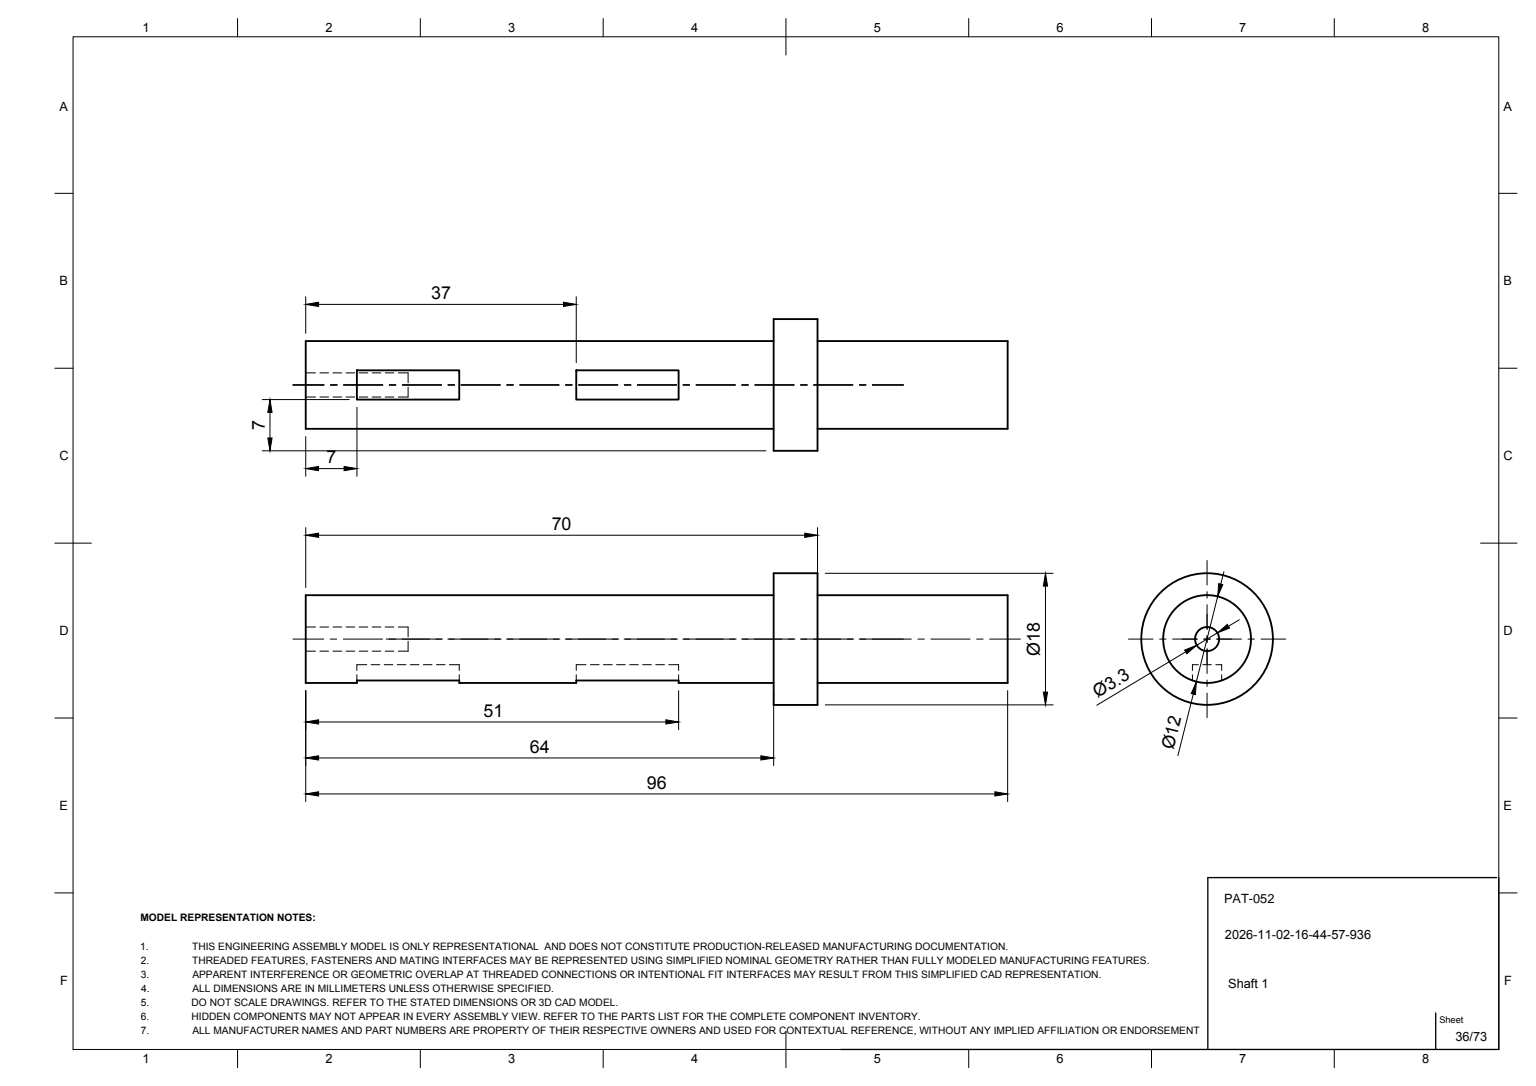
ISO-10303-21;
HEADER;
/* Generated by software containing ST-Developer
 * from STEP Tools, Inc. (www.steptools.com) 
 */

FILE_DESCRIPTION(
/* description */ ('Hand-crank gear train demonstrator'),
/* implementation_level */ '2;1');

FILE_NAME(
/* name */ 'Shaft 1.step',
/* time_stamp */ '2026-10-28T03:22:13-07:00',
/* author */ (''),
/* organization */ (''),
/* preprocessor_version */ 'ST-DEVELOPER v20.2',
/* originating_system */ 'Autodesk Translation Framework v15.17.0.0',
/* authorisation */ '');

FILE_SCHEMA (('AUTOMOTIVE_DESIGN { 1 0 10303 214 3 1 1 }'));
ENDSEC;

DATA;
#10=MECHANICAL_DESIGN_GEOMETRIC_PRESENTATION_REPRESENTATION('',(#1232),#62758);
#1089=SHAPE_REPRESENTATION_RELATIONSHIP('SRR','None',#63064,#1153);
#1153=ADVANCED_BREP_SHAPE_REPRESENTATION('',(#1308),#62718);
#1232=STYLED_ITEM('',(#63462),#1308);
#1308=MANIFOLD_SOLID_BREP('Body1',#16415);
#1542=FACE_BOUND('',#3696,.T.);
#1543=FACE_BOUND('',#3698,.T.);
#1544=FACE_BOUND('',#3702,.T.);
#1545=FACE_BOUND('',#3703,.T.);
#1546=FACE_BOUND('',#3705,.T.);
#1883=PLANE('',#17977);
#1884=PLANE('',#17978);
#1885=PLANE('',#17979);
#1886=PLANE('',#17981);
#1887=PLANE('',#17982);
#1888=PLANE('',#17983);
#1889=PLANE('',#17985);
#1890=PLANE('',#17986);
#1891=PLANE('',#17988);
#1892=PLANE('',#17989);
#1893=PLANE('',#17990);
#1894=PLANE('',#17992);
#1895=PLANE('',#17995);
#1896=PLANE('',#18003);
#1897=PLANE('',#18004);
#2547=FACE_OUTER_BOUND('',#3683,.T.);
#2548=FACE_OUTER_BOUND('',#3684,.T.);
#2549=FACE_OUTER_BOUND('',#3685,.T.);
#2550=FACE_OUTER_BOUND('',#3686,.T.);
#2551=FACE_OUTER_BOUND('',#3687,.T.);
#2552=FACE_OUTER_BOUND('',#3688,.T.);
#2553=FACE_OUTER_BOUND('',#3689,.T.);
#2554=FACE_OUTER_BOUND('',#3690,.T.);
#2555=FACE_OUTER_BOUND('',#3691,.T.);
#2556=FACE_OUTER_BOUND('',#3692,.T.);
#2557=FACE_OUTER_BOUND('',#3693,.T.);
#2558=FACE_OUTER_BOUND('',#3694,.T.);
#2559=FACE_OUTER_BOUND('',#3695,.T.);
#2560=FACE_OUTER_BOUND('',#3697,.T.);
#2561=FACE_OUTER_BOUND('',#3699,.T.);
#2562=FACE_OUTER_BOUND('',#3700,.T.);
#2563=FACE_OUTER_BOUND('',#3701,.T.);
#2564=FACE_OUTER_BOUND('',#3704,.T.);
#2565=FACE_OUTER_BOUND('',#3706,.T.);
#3683=EDGE_LOOP('',(#12709,#12710,#12711,#12712));
#3684=EDGE_LOOP('',(#12713));
#3685=EDGE_LOOP('',(#12714,#12715,#12716,#12717));
#3686=EDGE_LOOP('',(#12718,#12719,#12720,#12721));
#3687=EDGE_LOOP('',(#12722,#12723,#12724,#12725));
#3688=EDGE_LOOP('',(#12726,#12727,#12728,#12729));
#3689=EDGE_LOOP('',(#12730,#12731,#12732,#12733));
#3690=EDGE_LOOP('',(#12734,#12735,#12736,#12737));
#3691=EDGE_LOOP('',(#12738,#12739,#12740,#12741));
#3692=EDGE_LOOP('',(#12742,#12743,#12744,#12745));
#3693=EDGE_LOOP('',(#12746,#12747,#12748,#12749));
#3694=EDGE_LOOP('',(#12750,#12751,#12752,#12753));
#3695=EDGE_LOOP('',(#12754));
#3696=EDGE_LOOP('',(#12755));
#3697=EDGE_LOOP('',(#12756));
#3698=EDGE_LOOP('',(#12757));
#3699=EDGE_LOOP('',(#12758,#12759,#12760,#12761));
#3700=EDGE_LOOP('',(#12762,#12763,#12764,#12765));
#3701=EDGE_LOOP('',(#12766,#12767,#12768,#12769));
#3702=EDGE_LOOP('',(#12770,#12771,#12772,#12773));
#3703=EDGE_LOOP('',(#12774,#12775,#12776,#12777));
#3704=EDGE_LOOP('',(#12778));
#3705=EDGE_LOOP('',(#12779));
#3706=EDGE_LOOP('',(#12780));
#4843=LINE('',#25989,#5975);
#4844=LINE('',#25995,#5976);
#4845=LINE('',#25997,#5977);
#4846=LINE('',#25999,#5978);
#4847=LINE('',#26000,#5979);
#4848=LINE('',#26005,#5980);
#4849=LINE('',#26006,#5981);
#4850=LINE('',#26009,#5982);
#4851=LINE('',#26011,#5983);
#4852=LINE('',#26012,#5984);
#4853=LINE('',#26014,#5985);
#4854=LINE('',#26020,#5986);
#4855=LINE('',#26022,#5987);
#4856=LINE('',#26024,#5988);
#4857=LINE('',#26025,#5989);
#4858=LINE('',#26030,#5990);
#4859=LINE('',#26031,#5991);
#4860=LINE('',#26034,#5992);
#4861=LINE('',#26036,#5993);
#4862=LINE('',#26037,#5994);
#4863=LINE('',#26039,#5995);
#4864=LINE('',#26053,#5996);
#4865=LINE('',#26056,#5997);
#4866=LINE('',#26061,#5998);
#5975=VECTOR('',#21024,0.165);
#5976=VECTOR('',#21031,1.);
#5977=VECTOR('',#21032,1.);
#5978=VECTOR('',#21033,1.);
#5979=VECTOR('',#21034,1.);
#5980=VECTOR('',#21039,1.);
#5981=VECTOR('',#21040,1.);
#5982=VECTOR('',#21043,1.);
#5983=VECTOR('',#21044,1.);
#5984=VECTOR('',#21045,1.);
#5985=VECTOR('',#21048,1.);
#5986=VECTOR('',#21055,1.);
#5987=VECTOR('',#21056,1.);
#5988=VECTOR('',#21057,1.);
#5989=VECTOR('',#21058,1.);
#5990=VECTOR('',#21063,1.);
#5991=VECTOR('',#21064,1.);
#5992=VECTOR('',#21067,1.);
#5993=VECTOR('',#21068,1.);
#5994=VECTOR('',#21069,1.);
#5995=VECTOR('',#21072,1.);
#5996=VECTOR('',#21091,0.9);
#5997=VECTOR('',#21094,0.6);
#5998=VECTOR('',#21101,0.6);
#6898=CIRCLE('',#17975,0.165);
#6899=CIRCLE('',#17976,0.165);
#6900=CIRCLE('',#17980,0.6);
#6901=CIRCLE('',#17984,0.6);
#6902=CIRCLE('',#17987,0.6);
#6903=CIRCLE('',#17991,0.6);
#6904=CIRCLE('',#17993,0.9);
#6905=CIRCLE('',#17994,0.6);
#6906=CIRCLE('',#17996,0.9);
#6907=CIRCLE('',#17997,0.6);
#6908=CIRCLE('',#18000,0.6);
#6909=CIRCLE('',#18002,0.6);
#7851=VERTEX_POINT('',#25986);
#7852=VERTEX_POINT('',#25988);
#7853=VERTEX_POINT('',#25993);
#7854=VERTEX_POINT('',#25994);
#7855=VERTEX_POINT('',#25996);
#7856=VERTEX_POINT('',#25998);
#7857=VERTEX_POINT('',#26002);
#7858=VERTEX_POINT('',#26004);
#7859=VERTEX_POINT('',#26008);
#7860=VERTEX_POINT('',#26010);
#7861=VERTEX_POINT('',#26018);
#7862=VERTEX_POINT('',#26019);
#7863=VERTEX_POINT('',#26021);
#7864=VERTEX_POINT('',#26023);
#7865=VERTEX_POINT('',#26027);
#7866=VERTEX_POINT('',#26029);
#7867=VERTEX_POINT('',#26033);
#7868=VERTEX_POINT('',#26035);
#7869=VERTEX_POINT('',#26043);
#7870=VERTEX_POINT('',#26045);
#7871=VERTEX_POINT('',#26048);
#7872=VERTEX_POINT('',#26050);
#7873=VERTEX_POINT('',#26055);
#7874=VERTEX_POINT('',#26059);
#9606=EDGE_CURVE('',#7851,#7851,#6898,.T.);
#9607=EDGE_CURVE('',#7851,#7852,#4843,.T.);
#9608=EDGE_CURVE('',#7852,#7852,#6899,.T.);
#9609=EDGE_CURVE('',#7853,#7854,#4844,.T.);
#9610=EDGE_CURVE('',#7853,#7855,#4845,.T.);
#9611=EDGE_CURVE('',#7856,#7855,#4846,.T.);
#9612=EDGE_CURVE('',#7856,#7854,#4847,.T.);
#9613=EDGE_CURVE('',#7854,#7857,#6900,.T.);
#9614=EDGE_CURVE('',#7858,#7856,#4848,.T.);
#9615=EDGE_CURVE('',#7857,#7858,#4849,.T.);
#9616=EDGE_CURVE('',#7857,#7859,#4850,.T.);
#9617=EDGE_CURVE('',#7858,#7860,#4851,.T.);
#9618=EDGE_CURVE('',#7860,#7859,#4852,.T.);
#9619=EDGE_CURVE('',#7855,#7860,#4853,.T.);
#9620=EDGE_CURVE('',#7859,#7853,#6901,.T.);
#9621=EDGE_CURVE('',#7861,#7862,#4854,.T.);
#9622=EDGE_CURVE('',#7861,#7863,#4855,.T.);
#9623=EDGE_CURVE('',#7864,#7863,#4856,.T.);
#9624=EDGE_CURVE('',#7864,#7862,#4857,.T.);
#9625=EDGE_CURVE('',#7862,#7865,#6902,.T.);
#9626=EDGE_CURVE('',#7866,#7864,#4858,.T.);
#9627=EDGE_CURVE('',#7865,#7866,#4859,.T.);
#9628=EDGE_CURVE('',#7865,#7867,#4860,.T.);
#9629=EDGE_CURVE('',#7866,#7868,#4861,.T.);
#9630=EDGE_CURVE('',#7868,#7867,#4862,.T.);
#9631=EDGE_CURVE('',#7863,#7868,#4863,.T.);
#9632=EDGE_CURVE('',#7867,#7861,#6903,.T.);
#9633=EDGE_CURVE('',#7869,#7869,#6904,.T.);
#9634=EDGE_CURVE('',#7870,#7870,#6905,.T.);
#9635=EDGE_CURVE('',#7871,#7871,#6906,.T.);
#9636=EDGE_CURVE('',#7872,#7872,#6907,.T.);
#9637=EDGE_CURVE('',#7869,#7871,#4864,.T.);
#9638=EDGE_CURVE('',#7872,#7873,#4865,.T.);
#9639=EDGE_CURVE('',#7873,#7873,#6908,.T.);
#9640=EDGE_CURVE('',#7874,#7874,#6909,.T.);
#9641=EDGE_CURVE('',#7874,#7870,#4866,.T.);
#12709=ORIENTED_EDGE('',*,*,#9606,.F.);
#12710=ORIENTED_EDGE('',*,*,#9607,.T.);
#12711=ORIENTED_EDGE('',*,*,#9608,.F.);
#12712=ORIENTED_EDGE('',*,*,#9607,.F.);
#12713=ORIENTED_EDGE('',*,*,#9606,.T.);
#12714=ORIENTED_EDGE('',*,*,#9609,.F.);
#12715=ORIENTED_EDGE('',*,*,#9610,.T.);
#12716=ORIENTED_EDGE('',*,*,#9611,.F.);
#12717=ORIENTED_EDGE('',*,*,#9612,.T.);
#12718=ORIENTED_EDGE('',*,*,#9613,.F.);
#12719=ORIENTED_EDGE('',*,*,#9612,.F.);
#12720=ORIENTED_EDGE('',*,*,#9614,.F.);
#12721=ORIENTED_EDGE('',*,*,#9615,.F.);
#12722=ORIENTED_EDGE('',*,*,#9616,.F.);
#12723=ORIENTED_EDGE('',*,*,#9615,.T.);
#12724=ORIENTED_EDGE('',*,*,#9617,.T.);
#12725=ORIENTED_EDGE('',*,*,#9618,.T.);
#12726=ORIENTED_EDGE('',*,*,#9614,.T.);
#12727=ORIENTED_EDGE('',*,*,#9611,.T.);
#12728=ORIENTED_EDGE('',*,*,#9619,.T.);
#12729=ORIENTED_EDGE('',*,*,#9617,.F.);
#12730=ORIENTED_EDGE('',*,*,#9620,.F.);
#12731=ORIENTED_EDGE('',*,*,#9618,.F.);
#12732=ORIENTED_EDGE('',*,*,#9619,.F.);
#12733=ORIENTED_EDGE('',*,*,#9610,.F.);
#12734=ORIENTED_EDGE('',*,*,#9621,.F.);
#12735=ORIENTED_EDGE('',*,*,#9622,.T.);
#12736=ORIENTED_EDGE('',*,*,#9623,.F.);
#12737=ORIENTED_EDGE('',*,*,#9624,.T.);
#12738=ORIENTED_EDGE('',*,*,#9625,.F.);
#12739=ORIENTED_EDGE('',*,*,#9624,.F.);
#12740=ORIENTED_EDGE('',*,*,#9626,.F.);
#12741=ORIENTED_EDGE('',*,*,#9627,.F.);
#12742=ORIENTED_EDGE('',*,*,#9628,.F.);
#12743=ORIENTED_EDGE('',*,*,#9627,.T.);
#12744=ORIENTED_EDGE('',*,*,#9629,.T.);
#12745=ORIENTED_EDGE('',*,*,#9630,.T.);
#12746=ORIENTED_EDGE('',*,*,#9626,.T.);
#12747=ORIENTED_EDGE('',*,*,#9623,.T.);
#12748=ORIENTED_EDGE('',*,*,#9631,.T.);
#12749=ORIENTED_EDGE('',*,*,#9629,.F.);
#12750=ORIENTED_EDGE('',*,*,#9632,.F.);
#12751=ORIENTED_EDGE('',*,*,#9630,.F.);
#12752=ORIENTED_EDGE('',*,*,#9631,.F.);
#12753=ORIENTED_EDGE('',*,*,#9622,.F.);
#12754=ORIENTED_EDGE('',*,*,#9633,.T.);
#12755=ORIENTED_EDGE('',*,*,#9634,.F.);
#12756=ORIENTED_EDGE('',*,*,#9635,.F.);
#12757=ORIENTED_EDGE('',*,*,#9636,.F.);
#12758=ORIENTED_EDGE('',*,*,#9633,.F.);
#12759=ORIENTED_EDGE('',*,*,#9637,.T.);
#12760=ORIENTED_EDGE('',*,*,#9635,.T.);
#12761=ORIENTED_EDGE('',*,*,#9637,.F.);
#12762=ORIENTED_EDGE('',*,*,#9636,.T.);
#12763=ORIENTED_EDGE('',*,*,#9638,.T.);
#12764=ORIENTED_EDGE('',*,*,#9639,.T.);
#12765=ORIENTED_EDGE('',*,*,#9638,.F.);
#12766=ORIENTED_EDGE('',*,*,#9640,.F.);
#12767=ORIENTED_EDGE('',*,*,#9641,.T.);
#12768=ORIENTED_EDGE('',*,*,#9634,.T.);
#12769=ORIENTED_EDGE('',*,*,#9641,.F.);
#12770=ORIENTED_EDGE('',*,*,#9616,.T.);
#12771=ORIENTED_EDGE('',*,*,#9620,.T.);
#12772=ORIENTED_EDGE('',*,*,#9609,.T.);
#12773=ORIENTED_EDGE('',*,*,#9613,.T.);
#12774=ORIENTED_EDGE('',*,*,#9628,.T.);
#12775=ORIENTED_EDGE('',*,*,#9632,.T.);
#12776=ORIENTED_EDGE('',*,*,#9621,.T.);
#12777=ORIENTED_EDGE('',*,*,#9625,.T.);
#12778=ORIENTED_EDGE('',*,*,#9640,.T.);
#12779=ORIENTED_EDGE('',*,*,#9608,.T.);
#12780=ORIENTED_EDGE('',*,*,#9639,.F.);
#15290=CYLINDRICAL_SURFACE('',#17974,0.165);
#15291=CYLINDRICAL_SURFACE('',#17998,0.9);
#15292=CYLINDRICAL_SURFACE('',#17999,0.6);
#15293=CYLINDRICAL_SURFACE('',#18001,0.6);
#15857=ADVANCED_FACE('',(#2547),#15290,.F.);
#15858=ADVANCED_FACE('',(#2548),#1883,.T.);
#15859=ADVANCED_FACE('',(#2549),#1884,.F.);
#15860=ADVANCED_FACE('',(#2550),#1885,.T.);
#15861=ADVANCED_FACE('',(#2551),#1886,.F.);
#15862=ADVANCED_FACE('',(#2552),#1887,.F.);
#15863=ADVANCED_FACE('',(#2553),#1888,.F.);
#15864=ADVANCED_FACE('',(#2554),#1889,.F.);
#15865=ADVANCED_FACE('',(#2555),#1890,.T.);
#15866=ADVANCED_FACE('',(#2556),#1891,.F.);
#15867=ADVANCED_FACE('',(#2557),#1892,.F.);
#15868=ADVANCED_FACE('',(#2558),#1893,.F.);
#15869=ADVANCED_FACE('',(#2559,#1542),#1894,.T.);
#15870=ADVANCED_FACE('',(#2560,#1543),#1895,.F.);
#15871=ADVANCED_FACE('',(#2561),#15291,.T.);
#15872=ADVANCED_FACE('',(#2562),#15292,.T.);
#15873=ADVANCED_FACE('',(#2563,#1544,#1545),#15293,.T.);
#15874=ADVANCED_FACE('',(#2564,#1546),#1896,.T.);
#15875=ADVANCED_FACE('',(#2565),#1897,.F.);
#16415=CLOSED_SHELL('',(#15857,#15858,#15859,#15860,#15861,#15862,#15863,
#15864,#15865,#15866,#15867,#15868,#15869,#15870,#15871,#15872,#15873,#15874,
#15875));
#17973=AXIS2_PLACEMENT_3D('',#25984,#21018,#21019);
#17974=AXIS2_PLACEMENT_3D('',#25985,#21020,#21021);
#17975=AXIS2_PLACEMENT_3D('',#25987,#21022,#21023);
#17976=AXIS2_PLACEMENT_3D('',#25990,#21025,#21026);
#17977=AXIS2_PLACEMENT_3D('',#25991,#21027,#21028);
#17978=AXIS2_PLACEMENT_3D('',#25992,#21029,#21030);
#17979=AXIS2_PLACEMENT_3D('',#26001,#21035,#21036);
#17980=AXIS2_PLACEMENT_3D('',#26003,#21037,#21038);
#17981=AXIS2_PLACEMENT_3D('',#26007,#21041,#21042);
#17982=AXIS2_PLACEMENT_3D('',#26013,#21046,#21047);
#17983=AXIS2_PLACEMENT_3D('',#26015,#21049,#21050);
#17984=AXIS2_PLACEMENT_3D('',#26016,#21051,#21052);
#17985=AXIS2_PLACEMENT_3D('',#26017,#21053,#21054);
#17986=AXIS2_PLACEMENT_3D('',#26026,#21059,#21060);
#17987=AXIS2_PLACEMENT_3D('',#26028,#21061,#21062);
#17988=AXIS2_PLACEMENT_3D('',#26032,#21065,#21066);
#17989=AXIS2_PLACEMENT_3D('',#26038,#21070,#21071);
#17990=AXIS2_PLACEMENT_3D('',#26040,#21073,#21074);
#17991=AXIS2_PLACEMENT_3D('',#26041,#21075,#21076);
#17992=AXIS2_PLACEMENT_3D('',#26042,#21077,#21078);
#17993=AXIS2_PLACEMENT_3D('',#26044,#21079,#21080);
#17994=AXIS2_PLACEMENT_3D('',#26046,#21081,#21082);
#17995=AXIS2_PLACEMENT_3D('',#26047,#21083,#21084);
#17996=AXIS2_PLACEMENT_3D('',#26049,#21085,#21086);
#17997=AXIS2_PLACEMENT_3D('',#26051,#21087,#21088);
#17998=AXIS2_PLACEMENT_3D('',#26052,#21089,#21090);
#17999=AXIS2_PLACEMENT_3D('',#26054,#21092,#21093);
#18000=AXIS2_PLACEMENT_3D('',#26057,#21095,#21096);
#18001=AXIS2_PLACEMENT_3D('',#26058,#21097,#21098);
#18002=AXIS2_PLACEMENT_3D('',#26060,#21099,#21100);
#18003=AXIS2_PLACEMENT_3D('',#26062,#21102,#21103);
#18004=AXIS2_PLACEMENT_3D('',#26063,#21104,#21105);
#21018=DIRECTION('axis',(0.,0.,1.));
#21019=DIRECTION('refdir',(1.,0.,0.));
#21020=DIRECTION('center_axis',(0.,1.,0.));
#21021=DIRECTION('ref_axis',(1.,0.,0.));
#21022=DIRECTION('center_axis',(0.,1.,0.));
#21023=DIRECTION('ref_axis',(1.,0.,0.));
#21024=DIRECTION('',(0.,1.,0.));
#21025=DIRECTION('center_axis',(0.,-1.,0.));
#21026=DIRECTION('ref_axis',(1.,0.,0.));
#21027=DIRECTION('center_axis',(0.,1.,0.));
#21028=DIRECTION('ref_axis',(1.,0.,0.));
#21029=DIRECTION('center_axis',(-1.,0.,0.));
#21030=DIRECTION('ref_axis',(0.,0.,1.));
#21031=DIRECTION('',(0.,-1.,0.));
#21032=DIRECTION('',(0.,0.,1.));
#21033=DIRECTION('',(0.,1.,0.));
#21034=DIRECTION('',(0.,0.,-1.));
#21035=DIRECTION('center_axis',(0.,1.,0.));
#21036=DIRECTION('ref_axis',(1.,0.,0.));
#21037=DIRECTION('center_axis',(0.,-1.,0.));
#21038=DIRECTION('ref_axis',(1.,0.,0.));
#21039=DIRECTION('',(-1.,0.,0.));
#21040=DIRECTION('',(0.,0.,1.));
#21041=DIRECTION('center_axis',(1.,0.,0.));
#21042=DIRECTION('ref_axis',(0.,0.,-1.));
#21043=DIRECTION('',(0.,1.,0.));
#21044=DIRECTION('',(0.,1.,0.));
#21045=DIRECTION('',(0.,0.,-1.));
#21046=DIRECTION('center_axis',(0.,0.,1.));
#21047=DIRECTION('ref_axis',(1.,0.,0.));
#21048=DIRECTION('',(1.,0.,0.));
#21049=DIRECTION('center_axis',(0.,1.,0.));
#21050=DIRECTION('ref_axis',(0.,0.,1.));
#21051=DIRECTION('center_axis',(0.,1.,0.));
#21052=DIRECTION('ref_axis',(1.,0.,0.));
#21053=DIRECTION('center_axis',(-1.,0.,0.));
#21054=DIRECTION('ref_axis',(0.,0.,1.));
#21055=DIRECTION('',(0.,-1.,0.));
#21056=DIRECTION('',(0.,0.,1.));
#21057=DIRECTION('',(0.,1.,0.));
#21058=DIRECTION('',(0.,0.,-1.));
#21059=DIRECTION('center_axis',(0.,1.,0.));
#21060=DIRECTION('ref_axis',(1.,0.,0.));
#21061=DIRECTION('center_axis',(0.,-1.,0.));
#21062=DIRECTION('ref_axis',(1.,0.,0.));
#21063=DIRECTION('',(-1.,0.,0.));
#21064=DIRECTION('',(0.,0.,1.));
#21065=DIRECTION('center_axis',(1.,0.,0.));
#21066=DIRECTION('ref_axis',(0.,0.,-1.));
#21067=DIRECTION('',(0.,1.,0.));
#21068=DIRECTION('',(0.,1.,0.));
#21069=DIRECTION('',(0.,0.,-1.));
#21070=DIRECTION('center_axis',(0.,0.,1.));
#21071=DIRECTION('ref_axis',(1.,0.,0.));
#21072=DIRECTION('',(1.,0.,0.));
#21073=DIRECTION('center_axis',(0.,1.,0.));
#21074=DIRECTION('ref_axis',(0.,0.,1.));
#21075=DIRECTION('center_axis',(0.,1.,0.));
#21076=DIRECTION('ref_axis',(1.,0.,0.));
#21077=DIRECTION('center_axis',(0.,1.,0.));
#21078=DIRECTION('ref_axis',(1.,0.,0.));
#21079=DIRECTION('center_axis',(0.,1.,0.));
#21080=DIRECTION('ref_axis',(1.,0.,0.));
#21081=DIRECTION('center_axis',(0.,1.,0.));
#21082=DIRECTION('ref_axis',(1.,0.,0.));
#21083=DIRECTION('center_axis',(0.,1.,0.));
#21084=DIRECTION('ref_axis',(1.,0.,0.));
#21085=DIRECTION('center_axis',(0.,1.,0.));
#21086=DIRECTION('ref_axis',(1.,0.,0.));
#21087=DIRECTION('center_axis',(0.,-1.,0.));
#21088=DIRECTION('ref_axis',(1.,0.,0.));
#21089=DIRECTION('center_axis',(0.,1.,0.));
#21090=DIRECTION('ref_axis',(1.,0.,0.));
#21091=DIRECTION('',(0.,-1.,0.));
#21092=DIRECTION('center_axis',(0.,1.,0.));
#21093=DIRECTION('ref_axis',(1.,0.,0.));
#21094=DIRECTION('',(0.,-1.,0.));
#21095=DIRECTION('center_axis',(0.,1.,0.));
#21096=DIRECTION('ref_axis',(1.,0.,0.));
#21097=DIRECTION('center_axis',(0.,1.,0.));
#21098=DIRECTION('ref_axis',(1.,0.,0.));
#21099=DIRECTION('center_axis',(0.,1.,0.));
#21100=DIRECTION('ref_axis',(1.,0.,0.));
#21101=DIRECTION('',(0.,-1.,0.));
#21102=DIRECTION('center_axis',(0.,1.,0.));
#21103=DIRECTION('ref_axis',(1.,0.,0.));
#21104=DIRECTION('center_axis',(0.,1.,0.));
#21105=DIRECTION('ref_axis',(1.,0.,0.));
#25984=CARTESIAN_POINT('',(0.,0.,0.));
#25985=CARTESIAN_POINT('Origin',(0.,4.6,9.));
#25986=CARTESIAN_POINT('',(-0.165,4.6,9.));
#25987=CARTESIAN_POINT('Origin',(0.,4.6,9.));
#25988=CARTESIAN_POINT('',(-0.165,6.,9.));
#25989=CARTESIAN_POINT('',(-0.165,4.6,9.));
#25990=CARTESIAN_POINT('Origin',(0.,6.,9.));
#25991=CARTESIAN_POINT('Origin',(0.,4.6,9.));
#25992=CARTESIAN_POINT('Origin',(-0.2,3.9,8.3));
#25993=CARTESIAN_POINT('',(-0.2,5.3,8.43431457505076));
#25994=CARTESIAN_POINT('',(-0.2,3.9,8.43431457505076));
#25995=CARTESIAN_POINT('',(-0.2,-3.6,8.43431457505076));
#25996=CARTESIAN_POINT('',(-0.2,5.3,8.65));
#25997=CARTESIAN_POINT('',(-0.2,5.3,8.65));
#25998=CARTESIAN_POINT('',(-0.2,3.9,8.65));
#25999=CARTESIAN_POINT('',(-0.2,3.9,8.65));
#26000=CARTESIAN_POINT('',(-0.2,3.9,8.65));
#26001=CARTESIAN_POINT('Origin',(0.,3.9,8.475));
#26002=CARTESIAN_POINT('',(0.2,3.9,8.43431457505076));
#26003=CARTESIAN_POINT('Origin',(0.,3.9,9.));
#26004=CARTESIAN_POINT('',(0.2,3.9,8.65));
#26005=CARTESIAN_POINT('',(0.2,3.9,8.65));
#26006=CARTESIAN_POINT('',(0.2,3.9,8.3));
#26007=CARTESIAN_POINT('Origin',(0.2,3.9,8.65));
#26008=CARTESIAN_POINT('',(0.2,5.3,8.43431457505076));
#26009=CARTESIAN_POINT('',(0.2,-3.6,8.43431457505076));
#26010=CARTESIAN_POINT('',(0.2,5.3,8.65));
#26011=CARTESIAN_POINT('',(0.2,3.9,8.65));
#26012=CARTESIAN_POINT('',(0.2,5.3,8.3));
#26013=CARTESIAN_POINT('Origin',(-0.2,3.9,8.65));
#26014=CARTESIAN_POINT('',(0.2,5.3,8.65));
#26015=CARTESIAN_POINT('Origin',(0.,5.3,8.475));
#26016=CARTESIAN_POINT('Origin',(0.,5.3,9.));
#26017=CARTESIAN_POINT('Origin',(-0.2,0.9,7.8));
#26018=CARTESIAN_POINT('',(-0.2,2.3,8.43431457505076));
#26019=CARTESIAN_POINT('',(-0.2,0.9,8.43431457505076));
#26020=CARTESIAN_POINT('',(-0.2,-3.6,8.43431457505076));
#26021=CARTESIAN_POINT('',(-0.2,2.3,8.65));
#26022=CARTESIAN_POINT('',(-0.2,2.3,8.65));
#26023=CARTESIAN_POINT('',(-0.2,0.9,8.65));
#26024=CARTESIAN_POINT('',(-0.2,0.9,8.65));
#26025=CARTESIAN_POINT('',(-0.2,0.9,8.65));
#26026=CARTESIAN_POINT('Origin',(0.,0.9,8.225));
#26027=CARTESIAN_POINT('',(0.2,0.9,8.43431457505076));
#26028=CARTESIAN_POINT('Origin',(0.,0.9,9.));
#26029=CARTESIAN_POINT('',(0.2,0.9,8.65));
#26030=CARTESIAN_POINT('',(0.2,0.9,8.65));
#26031=CARTESIAN_POINT('',(0.2,0.9,7.8));
#26032=CARTESIAN_POINT('Origin',(0.2,0.9,8.65));
#26033=CARTESIAN_POINT('',(0.2,2.3,8.43431457505076));
#26034=CARTESIAN_POINT('',(0.2,-3.6,8.43431457505076));
#26035=CARTESIAN_POINT('',(0.2,2.3,8.65));
#26036=CARTESIAN_POINT('',(0.2,0.9,8.65));
#26037=CARTESIAN_POINT('',(0.2,2.3,7.8));
#26038=CARTESIAN_POINT('Origin',(-0.2,0.9,8.65));
#26039=CARTESIAN_POINT('',(0.2,2.3,8.65));
#26040=CARTESIAN_POINT('Origin',(0.,2.3,8.225));
#26041=CARTESIAN_POINT('Origin',(0.,2.3,9.));
#26042=CARTESIAN_POINT('Origin',(0.,-0.4,9.));
#26043=CARTESIAN_POINT('',(-0.9,-0.4,9.));
#26044=CARTESIAN_POINT('Origin',(0.,-0.4,9.));
#26045=CARTESIAN_POINT('',(-0.6,-0.4,9.));
#26046=CARTESIAN_POINT('Origin',(0.,-0.4,9.));
#26047=CARTESIAN_POINT('Origin',(0.,-1.,9.));
#26048=CARTESIAN_POINT('',(-0.9,-1.,9.));
#26049=CARTESIAN_POINT('Origin',(0.,-1.,9.));
#26050=CARTESIAN_POINT('',(-0.6,-1.,9.));
#26051=CARTESIAN_POINT('Origin',(0.,-1.,9.));
#26052=CARTESIAN_POINT('Origin',(0.,-1.,9.));
#26053=CARTESIAN_POINT('',(-0.9,-1.,9.));
#26054=CARTESIAN_POINT('Origin',(0.,-3.6,9.));
#26055=CARTESIAN_POINT('',(-0.6,-3.6,9.));
#26056=CARTESIAN_POINT('',(-0.6,-3.6,9.));
#26057=CARTESIAN_POINT('Origin',(0.,-3.6,9.));
#26058=CARTESIAN_POINT('Origin',(0.,-3.6,9.));
#26059=CARTESIAN_POINT('',(-0.6,6.,9.));
#26060=CARTESIAN_POINT('Origin',(0.,6.,9.));
#26061=CARTESIAN_POINT('',(-0.6,-3.6,9.));
#26062=CARTESIAN_POINT('Origin',(0.,6.,9.));
#26063=CARTESIAN_POINT('Origin',(0.,-3.6,9.));
#62644=UNCERTAINTY_MEASURE_WITH_UNIT(LENGTH_MEASURE(0.001),#62759,
'DISTANCE_ACCURACY_VALUE',
'Maximum model space distance between geometric entities at asserted c
onnectivities');
#62684=UNCERTAINTY_MEASURE_WITH_UNIT(LENGTH_MEASURE(0.001),#62759,
'DISTANCE_ACCURACY_VALUE',
'Maximum model space distance between geometric entities at asserted c
onnectivities');
#62718=(
GEOMETRIC_REPRESENTATION_CONTEXT(3)
GLOBAL_UNCERTAINTY_ASSIGNED_CONTEXT((#62644))
GLOBAL_UNIT_ASSIGNED_CONTEXT((#62759,#62761,#62762))
REPRESENTATION_CONTEXT('','3D')
);
#62758=(
GEOMETRIC_REPRESENTATION_CONTEXT(3)
GLOBAL_UNCERTAINTY_ASSIGNED_CONTEXT((#62684))
GLOBAL_UNIT_ASSIGNED_CONTEXT((#62759,#62761,#62762))
REPRESENTATION_CONTEXT('','3D')
);
#62759=(
LENGTH_UNIT()
NAMED_UNIT(*)
SI_UNIT(.CENTI.,.METRE.)
);
#62761=(
NAMED_UNIT(*)
PLANE_ANGLE_UNIT()
SI_UNIT($,.RADIAN.)
);
#62762=(
NAMED_UNIT(*)
SI_UNIT($,.STERADIAN.)
SOLID_ANGLE_UNIT()
);
#62796=SHAPE_DEFINITION_REPRESENTATION(#62879,#63064);
#62879=PRODUCT_DEFINITION_SHAPE('',$,#63138);
#63064=SHAPE_REPRESENTATION('',(#17973),#62718);
#63104=PRODUCT_DEFINITION_CONTEXT('part definition',#63325,'design');
#63138=PRODUCT_DEFINITION('Shaft 1','Shaft 1',#63211,#63104);
#63211=PRODUCT_DEFINITION_FORMATION('',$,#63360);
#63325=APPLICATION_CONTEXT(
'Core Data for Automotive Mechanical Design Process');
#63326=PRODUCT_CONTEXT('part definition',#63325,'mechanical');
#63360=PRODUCT('Shaft 1','Shaft 1','Shaft 1',(#63326));
#63456=COLOUR_RGB('Grey',0.48,0.52,0.57);
#63457=FILL_AREA_STYLE_COLOUR('',#63456);
#63458=FILL_AREA_STYLE('',(#63457));
#63459=SURFACE_STYLE_FILL_AREA(#63458);
#63460=SURFACE_SIDE_STYLE('',(#63459));
#63461=SURFACE_STYLE_USAGE(.BOTH.,#63460);
#63462=PRESENTATION_STYLE_ASSIGNMENT((#63461));
ENDSEC;
END-ISO-10303-21;
